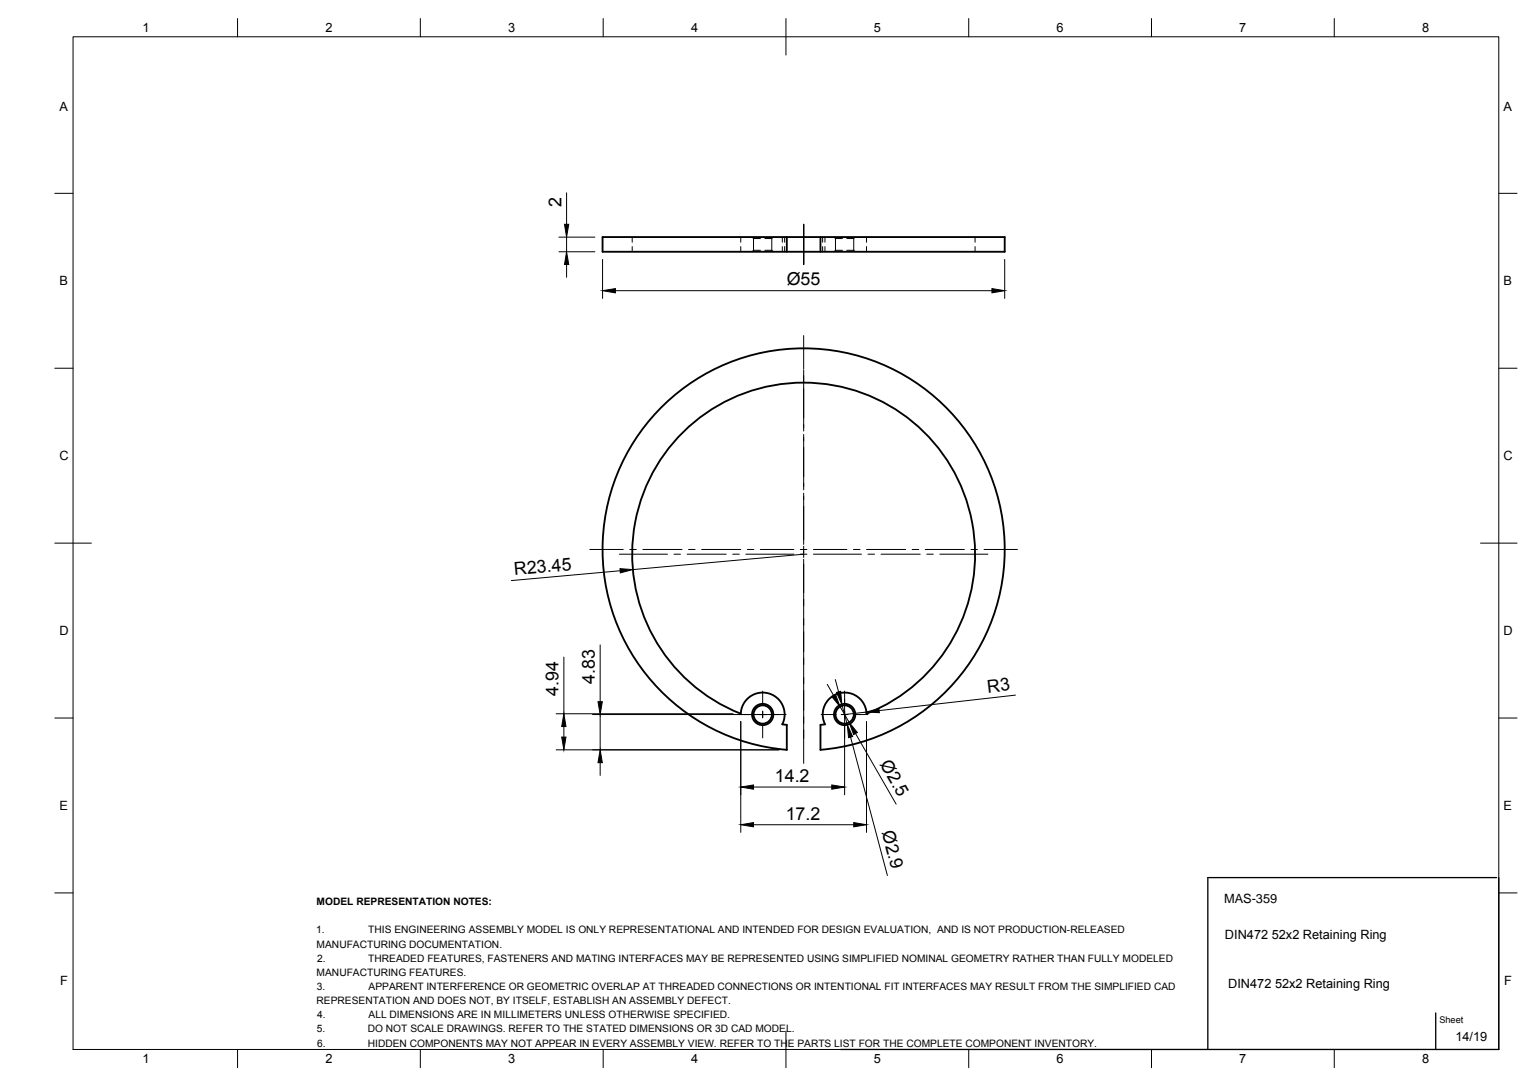
ISO-10303-21;
HEADER;
/* Generated by software containing ST-Developer
 * from STEP Tools, Inc. (www.steptools.com) 
 */

FILE_DESCRIPTION(
/* description */ (''),
/* implementation_level */ '2;1');

FILE_NAME(
/* name */ 'DIN472 52x2 Retaining Ring.step',
/* time_stamp */ '2026-10-15T14:25:16-07:00',
/* author */ (''),
/* organization */ (''),
/* preprocessor_version */ 'ST-DEVELOPER v20.2',
/* originating_system */ 'Autodesk Translation Framework v15.15.0.0',
/* authorisation */ '');

FILE_SCHEMA (('AUTOMOTIVE_DESIGN { 1 0 10303 214 3 1 1 }'));
ENDSEC;

DATA;
#10=MECHANICAL_DESIGN_GEOMETRIC_PRESENTATION_REPRESENTATION('',(#337),#86429);
#301=SHAPE_REPRESENTATION_RELATIONSHIP('SRR','None',#86516,#319);
#319=ADVANCED_BREP_SHAPE_REPRESENTATION('',(#355),#86425);
#337=STYLED_ITEM('',(#86615),#355);
#355=MANIFOLD_SOLID_BREP('Body1',#15627);
#1336=CONICAL_SURFACE('',#17085,0.135,0.785398163397449);
#1337=CONICAL_SURFACE('',#17098,0.135,0.785398163397448);
#1338=CONICAL_SURFACE('',#17108,0.135,0.785398163397449);
#1339=CONICAL_SURFACE('',#17112,0.135,0.785398163397448);
#1551=CYLINDRICAL_SURFACE('',#17088,0.125);
#1552=CYLINDRICAL_SURFACE('',#17110,0.125);
#1553=CYLINDRICAL_SURFACE('',#17115,2.345);
#1554=CYLINDRICAL_SURFACE('',#17116,0.3);
#1555=CYLINDRICAL_SURFACE('',#17117,2.345);
#1556=CYLINDRICAL_SURFACE('',#17118,0.3);
#1557=CYLINDRICAL_SURFACE('',#17119,2.345);
#1558=CYLINDRICAL_SURFACE('',#17120,2.75);
#1742=FACE_BOUND('',#4166,.T.);
#1743=FACE_BOUND('',#4167,.T.);
#1744=FACE_BOUND('',#4170,.T.);
#1745=FACE_BOUND('',#4171,.T.);
#2318=CIRCLE('',#17086,0.125);
#2319=CIRCLE('',#17087,0.145);
#2320=CIRCLE('',#17089,0.125);
#2321=CIRCLE('',#17091,2.75);
#2322=CIRCLE('',#17092,2.345);
#2323=CIRCLE('',#17093,0.3);
#2324=CIRCLE('',#17094,2.345);
#2325=CIRCLE('',#17095,0.3);
#2326=CIRCLE('',#17096,2.345);
#2327=CIRCLE('',#17097,0.145);
#2328=CIRCLE('',#17099,0.145);
#2329=CIRCLE('',#17101,2.345);
#2330=CIRCLE('',#17102,0.3);
#2331=CIRCLE('',#17103,2.345);
#2332=CIRCLE('',#17104,0.3);
#2333=CIRCLE('',#17105,2.345);
#2334=CIRCLE('',#17106,2.75);
#2335=CIRCLE('',#17107,0.145);
#2336=CIRCLE('',#17109,0.125);
#2337=CIRCLE('',#17111,0.125);
#3151=FACE_OUTER_BOUND('',#4163,.T.);
#3152=FACE_OUTER_BOUND('',#4164,.T.);
#3153=FACE_OUTER_BOUND('',#4165,.T.);
#3154=FACE_OUTER_BOUND('',#4168,.T.);
#3155=FACE_OUTER_BOUND('',#4169,.T.);
#3156=FACE_OUTER_BOUND('',#4172,.T.);
#3157=FACE_OUTER_BOUND('',#4173,.T.);
#3158=FACE_OUTER_BOUND('',#4174,.T.);
#3159=FACE_OUTER_BOUND('',#4175,.T.);
#3160=FACE_OUTER_BOUND('',#4176,.T.);
#3161=FACE_OUTER_BOUND('',#4177,.T.);
#3162=FACE_OUTER_BOUND('',#4178,.T.);
#3163=FACE_OUTER_BOUND('',#4179,.T.);
#3164=FACE_OUTER_BOUND('',#4180,.T.);
#3165=FACE_OUTER_BOUND('',#4181,.T.);
#3166=FACE_OUTER_BOUND('',#4182,.T.);
#4163=EDGE_LOOP('',(#13717,#13718,#13719,#13720));
#4164=EDGE_LOOP('',(#13721,#13722,#13723,#13724));
#4165=EDGE_LOOP('',(#13725,#13726,#13727,#13728,#13729,#13730,#13731,#13732));
#4166=EDGE_LOOP('',(#13733));
#4167=EDGE_LOOP('',(#13734));
#4168=EDGE_LOOP('',(#13735,#13736,#13737,#13738));
#4169=EDGE_LOOP('',(#13739,#13740,#13741,#13742,#13743,#13744,#13745,#13746));
#4170=EDGE_LOOP('',(#13747));
#4171=EDGE_LOOP('',(#13748));
#4172=EDGE_LOOP('',(#13749,#13750,#13751,#13752));
#4173=EDGE_LOOP('',(#13753,#13754,#13755,#13756));
#4174=EDGE_LOOP('',(#13757,#13758,#13759,#13760));
#4175=EDGE_LOOP('',(#13761,#13762,#13763,#13764));
#4176=EDGE_LOOP('',(#13765,#13766,#13767,#13768));
#4177=EDGE_LOOP('',(#13769,#13770,#13771,#13772));
#4178=EDGE_LOOP('',(#13773,#13774,#13775,#13776));
#4179=EDGE_LOOP('',(#13777,#13778,#13779,#13780));
#4180=EDGE_LOOP('',(#13781,#13782,#13783,#13784));
#4181=EDGE_LOOP('',(#13785,#13786,#13787,#13788));
#4182=EDGE_LOOP('',(#13789,#13790,#13791,#13792));
#5049=LINE('',#66556,#5909);
#5050=LINE('',#66560,#5910);
#5051=LINE('',#66565,#5911);
#5052=LINE('',#66569,#5912);
#5053=LINE('',#66583,#5913);
#5054=LINE('',#66588,#5914);
#5055=LINE('',#66600,#5915);
#5056=LINE('',#66607,#5916);
#5057=LINE('',#66610,#5917);
#5058=LINE('',#66613,#5918);
#5059=LINE('',#66615,#5919);
#5060=LINE('',#66616,#5920);
#5061=LINE('',#66618,#5921);
#5062=LINE('',#66619,#5922);
#5063=LINE('',#66621,#5923);
#5064=LINE('',#66623,#5924);
#5065=LINE('',#66625,#5925);
#5066=LINE('',#66627,#5926);
#5909=VECTOR('',#20568,0.135);
#5910=VECTOR('',#20573,0.125);
#5911=VECTOR('',#20578,1.);
#5912=VECTOR('',#20581,1.);
#5913=VECTOR('',#20596,0.135);
#5914=VECTOR('',#20601,1.);
#5915=VECTOR('',#20612,1.);
#5916=VECTOR('',#20621,0.135);
#5917=VECTOR('',#20624,0.125);
#5918=VECTOR('',#20629,0.135);
#5919=VECTOR('',#20632,1.);
#5920=VECTOR('',#20633,1.);
#5921=VECTOR('',#20636,1.);
#5922=VECTOR('',#20637,1.);
#5923=VECTOR('',#20640,1.);
#5924=VECTOR('',#20643,1.);
#5925=VECTOR('',#20646,1.);
#5926=VECTOR('',#20649,1.);
#7266=VERTEX_POINT('',#66553);
#7267=VERTEX_POINT('',#66555);
#7268=VERTEX_POINT('',#66559);
#7269=VERTEX_POINT('',#66563);
#7270=VERTEX_POINT('',#66564);
#7271=VERTEX_POINT('',#66566);
#7272=VERTEX_POINT('',#66568);
#7273=VERTEX_POINT('',#66570);
#7274=VERTEX_POINT('',#66572);
#7275=VERTEX_POINT('',#66574);
#7276=VERTEX_POINT('',#66576);
#7277=VERTEX_POINT('',#66579);
#7278=VERTEX_POINT('',#66582);
#7279=VERTEX_POINT('',#66586);
#7280=VERTEX_POINT('',#66587);
#7281=VERTEX_POINT('',#66589);
#7282=VERTEX_POINT('',#66591);
#7283=VERTEX_POINT('',#66593);
#7284=VERTEX_POINT('',#66595);
#7285=VERTEX_POINT('',#66597);
#7286=VERTEX_POINT('',#66599);
#7287=VERTEX_POINT('',#66602);
#7288=VERTEX_POINT('',#66605);
#7289=VERTEX_POINT('',#66609);
#9480=EDGE_CURVE('',#7266,#7266,#2318,.T.);
#9481=EDGE_CURVE('',#7266,#7267,#5049,.T.);
#9482=EDGE_CURVE('',#7267,#7267,#2319,.T.);
#9483=EDGE_CURVE('',#7266,#7268,#5050,.T.);
#9484=EDGE_CURVE('',#7268,#7268,#2320,.T.);
#9485=EDGE_CURVE('',#7269,#7270,#5051,.T.);
#9486=EDGE_CURVE('',#7271,#7270,#2321,.T.);
#9487=EDGE_CURVE('',#7271,#7272,#5052,.T.);
#9488=EDGE_CURVE('',#7273,#7272,#2322,.T.);
#9489=EDGE_CURVE('',#7274,#7273,#2323,.T.);
#9490=EDGE_CURVE('',#7275,#7274,#2324,.T.);
#9491=EDGE_CURVE('',#7276,#7275,#2325,.T.);
#9492=EDGE_CURVE('',#7269,#7276,#2326,.T.);
#9493=EDGE_CURVE('',#7277,#7277,#2327,.T.);
#9494=EDGE_CURVE('',#7268,#7278,#5053,.T.);
#9495=EDGE_CURVE('',#7278,#7278,#2328,.T.);
#9496=EDGE_CURVE('',#7279,#7280,#5054,.T.);
#9497=EDGE_CURVE('',#7280,#7281,#2329,.T.);
#9498=EDGE_CURVE('',#7281,#7282,#2330,.T.);
#9499=EDGE_CURVE('',#7282,#7283,#2331,.T.);
#9500=EDGE_CURVE('',#7283,#7284,#2332,.T.);
#9501=EDGE_CURVE('',#7284,#7285,#2333,.T.);
#9502=EDGE_CURVE('',#7285,#7286,#5055,.T.);
#9503=EDGE_CURVE('',#7286,#7279,#2334,.T.);
#9504=EDGE_CURVE('',#7287,#7287,#2335,.T.);
#9505=EDGE_CURVE('',#7288,#7288,#2336,.T.);
#9506=EDGE_CURVE('',#7288,#7277,#5056,.T.);
#9507=EDGE_CURVE('',#7288,#7289,#5057,.T.);
#9508=EDGE_CURVE('',#7289,#7289,#2337,.T.);
#9509=EDGE_CURVE('',#7289,#7287,#5058,.T.);
#9510=EDGE_CURVE('',#7272,#7285,#5059,.T.);
#9511=EDGE_CURVE('',#7286,#7271,#5060,.T.);
#9512=EDGE_CURVE('',#7280,#7269,#5061,.T.);
#9513=EDGE_CURVE('',#7270,#7279,#5062,.T.);
#9514=EDGE_CURVE('',#7273,#7284,#5063,.T.);
#9515=EDGE_CURVE('',#7274,#7283,#5064,.T.);
#9516=EDGE_CURVE('',#7275,#7282,#5065,.T.);
#9517=EDGE_CURVE('',#7276,#7281,#5066,.T.);
#13717=ORIENTED_EDGE('',*,*,#9480,.T.);
#13718=ORIENTED_EDGE('',*,*,#9481,.T.);
#13719=ORIENTED_EDGE('',*,*,#9482,.T.);
#13720=ORIENTED_EDGE('',*,*,#9481,.F.);
#13721=ORIENTED_EDGE('',*,*,#9480,.F.);
#13722=ORIENTED_EDGE('',*,*,#9483,.T.);
#13723=ORIENTED_EDGE('',*,*,#9484,.F.);
#13724=ORIENTED_EDGE('',*,*,#9483,.F.);
#13725=ORIENTED_EDGE('',*,*,#9485,.T.);
#13726=ORIENTED_EDGE('',*,*,#9486,.F.);
#13727=ORIENTED_EDGE('',*,*,#9487,.T.);
#13728=ORIENTED_EDGE('',*,*,#9488,.F.);
#13729=ORIENTED_EDGE('',*,*,#9489,.F.);
#13730=ORIENTED_EDGE('',*,*,#9490,.F.);
#13731=ORIENTED_EDGE('',*,*,#9491,.F.);
#13732=ORIENTED_EDGE('',*,*,#9492,.F.);
#13733=ORIENTED_EDGE('',*,*,#9493,.F.);
#13734=ORIENTED_EDGE('',*,*,#9482,.F.);
#13735=ORIENTED_EDGE('',*,*,#9484,.T.);
#13736=ORIENTED_EDGE('',*,*,#9494,.T.);
#13737=ORIENTED_EDGE('',*,*,#9495,.T.);
#13738=ORIENTED_EDGE('',*,*,#9494,.F.);
#13739=ORIENTED_EDGE('',*,*,#9496,.T.);
#13740=ORIENTED_EDGE('',*,*,#9497,.T.);
#13741=ORIENTED_EDGE('',*,*,#9498,.T.);
#13742=ORIENTED_EDGE('',*,*,#9499,.T.);
#13743=ORIENTED_EDGE('',*,*,#9500,.T.);
#13744=ORIENTED_EDGE('',*,*,#9501,.T.);
#13745=ORIENTED_EDGE('',*,*,#9502,.T.);
#13746=ORIENTED_EDGE('',*,*,#9503,.T.);
#13747=ORIENTED_EDGE('',*,*,#9504,.F.);
#13748=ORIENTED_EDGE('',*,*,#9495,.F.);
#13749=ORIENTED_EDGE('',*,*,#9505,.T.);
#13750=ORIENTED_EDGE('',*,*,#9506,.T.);
#13751=ORIENTED_EDGE('',*,*,#9493,.T.);
#13752=ORIENTED_EDGE('',*,*,#9506,.F.);
#13753=ORIENTED_EDGE('',*,*,#9505,.F.);
#13754=ORIENTED_EDGE('',*,*,#9507,.T.);
#13755=ORIENTED_EDGE('',*,*,#9508,.F.);
#13756=ORIENTED_EDGE('',*,*,#9507,.F.);
#13757=ORIENTED_EDGE('',*,*,#9508,.T.);
#13758=ORIENTED_EDGE('',*,*,#9509,.T.);
#13759=ORIENTED_EDGE('',*,*,#9504,.T.);
#13760=ORIENTED_EDGE('',*,*,#9509,.F.);
#13761=ORIENTED_EDGE('',*,*,#9510,.F.);
#13762=ORIENTED_EDGE('',*,*,#9487,.F.);
#13763=ORIENTED_EDGE('',*,*,#9511,.F.);
#13764=ORIENTED_EDGE('',*,*,#9502,.F.);
#13765=ORIENTED_EDGE('',*,*,#9512,.F.);
#13766=ORIENTED_EDGE('',*,*,#9496,.F.);
#13767=ORIENTED_EDGE('',*,*,#9513,.F.);
#13768=ORIENTED_EDGE('',*,*,#9485,.F.);
#13769=ORIENTED_EDGE('',*,*,#9510,.T.);
#13770=ORIENTED_EDGE('',*,*,#9501,.F.);
#13771=ORIENTED_EDGE('',*,*,#9514,.F.);
#13772=ORIENTED_EDGE('',*,*,#9488,.T.);
#13773=ORIENTED_EDGE('',*,*,#9489,.T.);
#13774=ORIENTED_EDGE('',*,*,#9514,.T.);
#13775=ORIENTED_EDGE('',*,*,#9500,.F.);
#13776=ORIENTED_EDGE('',*,*,#9515,.F.);
#13777=ORIENTED_EDGE('',*,*,#9490,.T.);
#13778=ORIENTED_EDGE('',*,*,#9515,.T.);
#13779=ORIENTED_EDGE('',*,*,#9499,.F.);
#13780=ORIENTED_EDGE('',*,*,#9516,.F.);
#13781=ORIENTED_EDGE('',*,*,#9491,.T.);
#13782=ORIENTED_EDGE('',*,*,#9516,.T.);
#13783=ORIENTED_EDGE('',*,*,#9498,.F.);
#13784=ORIENTED_EDGE('',*,*,#9517,.F.);
#13785=ORIENTED_EDGE('',*,*,#9512,.T.);
#13786=ORIENTED_EDGE('',*,*,#9492,.T.);
#13787=ORIENTED_EDGE('',*,*,#9517,.T.);
#13788=ORIENTED_EDGE('',*,*,#9497,.F.);
#13789=ORIENTED_EDGE('',*,*,#9513,.T.);
#13790=ORIENTED_EDGE('',*,*,#9503,.F.);
#13791=ORIENTED_EDGE('',*,*,#9511,.T.);
#13792=ORIENTED_EDGE('',*,*,#9486,.T.);
#14709=PLANE('',#17090);
#14710=PLANE('',#17100);
#14711=PLANE('',#17113);
#14712=PLANE('',#17114);
#15507=ADVANCED_FACE('',(#3151),#1336,.F.);
#15508=ADVANCED_FACE('',(#3152),#1551,.F.);
#15509=ADVANCED_FACE('',(#3153,#1742,#1743),#14709,.F.);
#15510=ADVANCED_FACE('',(#3154),#1337,.F.);
#15511=ADVANCED_FACE('',(#3155,#1744,#1745),#14710,.T.);
#15512=ADVANCED_FACE('',(#3156),#1338,.F.);
#15513=ADVANCED_FACE('',(#3157),#1552,.F.);
#15514=ADVANCED_FACE('',(#3158),#1339,.F.);
#15515=ADVANCED_FACE('',(#3159),#14711,.F.);
#15516=ADVANCED_FACE('',(#3160),#14712,.F.);
#15517=ADVANCED_FACE('',(#3161),#1553,.F.);
#15518=ADVANCED_FACE('',(#3162),#1554,.T.);
#15519=ADVANCED_FACE('',(#3163),#1555,.F.);
#15520=ADVANCED_FACE('',(#3164),#1556,.T.);
#15521=ADVANCED_FACE('',(#3165),#1557,.F.);
#15522=ADVANCED_FACE('',(#3166),#1558,.T.);
#15627=CLOSED_SHELL('',(#15507,#15508,#15509,#15510,#15511,#15512,#15513,
#15514,#15515,#15516,#15517,#15518,#15519,#15520,#15521,#15522));
#17084=AXIS2_PLACEMENT_3D('',#66551,#20562,#20563);
#17085=AXIS2_PLACEMENT_3D('',#66552,#20564,#20565);
#17086=AXIS2_PLACEMENT_3D('',#66554,#20566,#20567);
#17087=AXIS2_PLACEMENT_3D('',#66557,#20569,#20570);
#17088=AXIS2_PLACEMENT_3D('',#66558,#20571,#20572);
#17089=AXIS2_PLACEMENT_3D('',#66561,#20574,#20575);
#17090=AXIS2_PLACEMENT_3D('',#66562,#20576,#20577);
#17091=AXIS2_PLACEMENT_3D('',#66567,#20579,#20580);
#17092=AXIS2_PLACEMENT_3D('',#66571,#20582,#20583);
#17093=AXIS2_PLACEMENT_3D('',#66573,#20584,#20585);
#17094=AXIS2_PLACEMENT_3D('',#66575,#20586,#20587);
#17095=AXIS2_PLACEMENT_3D('',#66577,#20588,#20589);
#17096=AXIS2_PLACEMENT_3D('',#66578,#20590,#20591);
#17097=AXIS2_PLACEMENT_3D('',#66580,#20592,#20593);
#17098=AXIS2_PLACEMENT_3D('',#66581,#20594,#20595);
#17099=AXIS2_PLACEMENT_3D('',#66584,#20597,#20598);
#17100=AXIS2_PLACEMENT_3D('',#66585,#20599,#20600);
#17101=AXIS2_PLACEMENT_3D('',#66590,#20602,#20603);
#17102=AXIS2_PLACEMENT_3D('',#66592,#20604,#20605);
#17103=AXIS2_PLACEMENT_3D('',#66594,#20606,#20607);
#17104=AXIS2_PLACEMENT_3D('',#66596,#20608,#20609);
#17105=AXIS2_PLACEMENT_3D('',#66598,#20610,#20611);
#17106=AXIS2_PLACEMENT_3D('',#66601,#20613,#20614);
#17107=AXIS2_PLACEMENT_3D('',#66603,#20615,#20616);
#17108=AXIS2_PLACEMENT_3D('',#66604,#20617,#20618);
#17109=AXIS2_PLACEMENT_3D('',#66606,#20619,#20620);
#17110=AXIS2_PLACEMENT_3D('',#66608,#20622,#20623);
#17111=AXIS2_PLACEMENT_3D('',#66611,#20625,#20626);
#17112=AXIS2_PLACEMENT_3D('',#66612,#20627,#20628);
#17113=AXIS2_PLACEMENT_3D('',#66614,#20630,#20631);
#17114=AXIS2_PLACEMENT_3D('',#66617,#20634,#20635);
#17115=AXIS2_PLACEMENT_3D('',#66620,#20638,#20639);
#17116=AXIS2_PLACEMENT_3D('',#66622,#20641,#20642);
#17117=AXIS2_PLACEMENT_3D('',#66624,#20644,#20645);
#17118=AXIS2_PLACEMENT_3D('',#66626,#20647,#20648);
#17119=AXIS2_PLACEMENT_3D('',#66628,#20650,#20651);
#17120=AXIS2_PLACEMENT_3D('',#66629,#20652,#20653);
#20562=DIRECTION('axis',(0.,0.,1.));
#20563=DIRECTION('refdir',(1.,0.,0.));
#20564=DIRECTION('center_axis',(0.,0.,-1.));
#20565=DIRECTION('ref_axis',(1.,0.,0.));
#20566=DIRECTION('center_axis',(0.,0.,1.));
#20567=DIRECTION('ref_axis',(1.,0.,0.));
#20568=DIRECTION('',(-0.707106781186548,8.65956056235494E-17,-0.707106781186547));
#20569=DIRECTION('center_axis',(0.,0.,-1.));
#20570=DIRECTION('ref_axis',(1.,0.,0.));
#20571=DIRECTION('center_axis',(0.,0.,1.));
#20572=DIRECTION('ref_axis',(1.,0.,0.));
#20573=DIRECTION('',(0.,0.,1.));
#20574=DIRECTION('center_axis',(0.,0.,-1.));
#20575=DIRECTION('ref_axis',(1.,0.,0.));
#20576=DIRECTION('center_axis',(0.,0.,1.));
#20577=DIRECTION('ref_axis',(1.,0.,0.));
#20578=DIRECTION('',(0.,1.,0.));
#20579=DIRECTION('center_axis',(0.,0.,1.));
#20580=DIRECTION('ref_axis',(1.,0.,0.));
#20581=DIRECTION('',(0.,-1.,0.));
#20582=DIRECTION('center_axis',(0.,0.,-1.));
#20583=DIRECTION('ref_axis',(1.,0.,0.));
#20584=DIRECTION('center_axis',(0.,0.,1.));
#20585=DIRECTION('ref_axis',(1.,0.,0.));
#20586=DIRECTION('center_axis',(0.,0.,-1.));
#20587=DIRECTION('ref_axis',(1.,0.,0.));
#20588=DIRECTION('center_axis',(0.,0.,1.));
#20589=DIRECTION('ref_axis',(1.,0.,0.));
#20590=DIRECTION('center_axis',(0.,0.,-1.));
#20591=DIRECTION('ref_axis',(1.,0.,0.));
#20592=DIRECTION('center_axis',(0.,0.,-1.));
#20593=DIRECTION('ref_axis',(1.,0.,0.));
#20594=DIRECTION('center_axis',(0.,0.,1.));
#20595=DIRECTION('ref_axis',(1.,0.,0.));
#20596=DIRECTION('',(-0.707106781186547,-8.65956056235493E-17,0.707106781186548));
#20597=DIRECTION('center_axis',(0.,0.,1.));
#20598=DIRECTION('ref_axis',(1.,0.,0.));
#20599=DIRECTION('center_axis',(0.,0.,1.));
#20600=DIRECTION('ref_axis',(1.,0.,0.));
#20601=DIRECTION('',(0.,-1.,0.));
#20602=DIRECTION('center_axis',(0.,0.,-1.));
#20603=DIRECTION('ref_axis',(1.,0.,0.));
#20604=DIRECTION('center_axis',(0.,0.,1.));
#20605=DIRECTION('ref_axis',(1.,0.,0.));
#20606=DIRECTION('center_axis',(0.,0.,-1.));
#20607=DIRECTION('ref_axis',(1.,0.,0.));
#20608=DIRECTION('center_axis',(0.,0.,1.));
#20609=DIRECTION('ref_axis',(1.,0.,0.));
#20610=DIRECTION('center_axis',(0.,0.,-1.));
#20611=DIRECTION('ref_axis',(1.,0.,0.));
#20612=DIRECTION('',(0.,1.,0.));
#20613=DIRECTION('center_axis',(0.,0.,1.));
#20614=DIRECTION('ref_axis',(1.,0.,0.));
#20615=DIRECTION('center_axis',(0.,0.,1.));
#20616=DIRECTION('ref_axis',(1.,0.,0.));
#20617=DIRECTION('center_axis',(0.,0.,-1.));
#20618=DIRECTION('ref_axis',(1.,0.,0.));
#20619=DIRECTION('center_axis',(0.,0.,1.));
#20620=DIRECTION('ref_axis',(1.,0.,0.));
#20621=DIRECTION('',(-0.707106781186548,8.65956056235494E-17,-0.707106781186547));
#20622=DIRECTION('center_axis',(0.,0.,1.));
#20623=DIRECTION('ref_axis',(1.,0.,0.));
#20624=DIRECTION('',(0.,0.,1.));
#20625=DIRECTION('center_axis',(0.,0.,-1.));
#20626=DIRECTION('ref_axis',(1.,0.,0.));
#20627=DIRECTION('center_axis',(0.,0.,1.));
#20628=DIRECTION('ref_axis',(1.,0.,0.));
#20629=DIRECTION('',(-0.707106781186547,-8.65956056235493E-17,0.707106781186548));
#20630=DIRECTION('center_axis',(-1.,0.,0.));
#20631=DIRECTION('ref_axis',(0.,-1.,0.));
#20632=DIRECTION('',(0.,0.,1.));
#20633=DIRECTION('',(0.,0.,-1.));
#20634=DIRECTION('center_axis',(1.,0.,0.));
#20635=DIRECTION('ref_axis',(0.,1.,0.));
#20636=DIRECTION('',(0.,0.,-1.));
#20637=DIRECTION('',(0.,0.,1.));
#20638=DIRECTION('center_axis',(0.,0.,1.));
#20639=DIRECTION('ref_axis',(1.,0.,0.));
#20640=DIRECTION('',(0.,0.,1.));
#20641=DIRECTION('center_axis',(0.,0.,1.));
#20642=DIRECTION('ref_axis',(1.,0.,0.));
#20643=DIRECTION('',(0.,0.,1.));
#20644=DIRECTION('center_axis',(0.,0.,1.));
#20645=DIRECTION('ref_axis',(-1.83697019872103E-16,-1.,0.));
#20646=DIRECTION('',(0.,0.,1.));
#20647=DIRECTION('center_axis',(0.,0.,1.));
#20648=DIRECTION('ref_axis',(-0.247524504876091,-0.96888163337213,0.));
#20649=DIRECTION('',(0.,0.,1.));
#20650=DIRECTION('center_axis',(0.,0.,1.));
#20651=DIRECTION('ref_axis',(1.,0.,0.));
#20652=DIRECTION('center_axis',(0.,0.,1.));
#20653=DIRECTION('ref_axis',(6.12323399573677E-17,-1.,0.));
#66551=CARTESIAN_POINT('',(0.,0.,0.));
#66552=CARTESIAN_POINT('Origin',(-0.56,2.257,0.01));
#66553=CARTESIAN_POINT('',(-0.685,2.257,0.02));
#66554=CARTESIAN_POINT('Origin',(-0.56,2.257,0.02));
#66555=CARTESIAN_POINT('',(-0.705,2.257,0.));
#66556=CARTESIAN_POINT('',(-0.695,2.257,0.01));
#66557=CARTESIAN_POINT('Origin',(-0.56,2.257,0.));
#66558=CARTESIAN_POINT('Origin',(-0.56,2.257,0.));
#66559=CARTESIAN_POINT('',(-0.685,2.257,0.18));
#66560=CARTESIAN_POINT('',(-0.685,2.257,0.));
#66561=CARTESIAN_POINT('Origin',(-0.56,2.257,0.18));
#66562=CARTESIAN_POINT('Origin',(0.,0.,0.));
#66563=CARTESIAN_POINT('',(0.23,2.39869342459544,0.));
#66564=CARTESIAN_POINT('',(0.23,2.74036493920062,0.));
#66565=CARTESIAN_POINT('',(0.23,0.9,0.));
#66566=CARTESIAN_POINT('',(-0.23,2.74036493920062,0.));
#66567=CARTESIAN_POINT('Origin',(0.,0.,0.));
#66568=CARTESIAN_POINT('',(-0.23,2.39869342459544,0.));
#66569=CARTESIAN_POINT('',(-0.23,1.45,0.));
#66570=CARTESIAN_POINT('',(-0.291967181462275,2.39175313794759,0.));
#66571=CARTESIAN_POINT('Origin',(0.,0.065,0.));
#66572=CARTESIAN_POINT('',(-0.859822464806605,2.24668062030488,0.));
#66573=CARTESIAN_POINT('Origin',(-0.56,2.257,0.));
#66574=CARTESIAN_POINT('',(0.859822464806605,2.24668062030488,0.));
#66575=CARTESIAN_POINT('Origin',(0.,0.065,0.));
#66576=CARTESIAN_POINT('',(0.291967181462275,2.39175313794759,0.));
#66577=CARTESIAN_POINT('Origin',(0.56,2.257,0.));
#66578=CARTESIAN_POINT('Origin',(0.,0.065,0.));
#66579=CARTESIAN_POINT('',(0.415,2.257,0.));
#66580=CARTESIAN_POINT('Origin',(0.56,2.257,0.));
#66581=CARTESIAN_POINT('Origin',(-0.56,2.257,0.19));
#66582=CARTESIAN_POINT('',(-0.705,2.257,0.2));
#66583=CARTESIAN_POINT('',(-0.695,2.257,0.19));
#66584=CARTESIAN_POINT('Origin',(-0.56,2.257,0.2));
#66585=CARTESIAN_POINT('Origin',(0.,0.,0.2));
#66586=CARTESIAN_POINT('',(0.23,2.74036493920062,0.2));
#66587=CARTESIAN_POINT('',(0.23,2.39869342459544,0.2));
#66588=CARTESIAN_POINT('',(0.23,0.9,0.2));
#66589=CARTESIAN_POINT('',(0.291967181462275,2.39175313794759,0.2));
#66590=CARTESIAN_POINT('Origin',(0.,0.065,0.2));
#66591=CARTESIAN_POINT('',(0.859822464806605,2.24668062030488,0.2));
#66592=CARTESIAN_POINT('Origin',(0.56,2.257,0.2));
#66593=CARTESIAN_POINT('',(-0.859822464806605,2.24668062030488,0.2));
#66594=CARTESIAN_POINT('Origin',(0.,0.065,0.2));
#66595=CARTESIAN_POINT('',(-0.291967181462275,2.39175313794759,0.2));
#66596=CARTESIAN_POINT('Origin',(-0.56,2.257,0.2));
#66597=CARTESIAN_POINT('',(-0.23,2.39869342459544,0.2));
#66598=CARTESIAN_POINT('Origin',(0.,0.065,0.2));
#66599=CARTESIAN_POINT('',(-0.23,2.74036493920062,0.2));
#66600=CARTESIAN_POINT('',(-0.23,1.45,0.2));
#66601=CARTESIAN_POINT('Origin',(0.,0.,0.2));
#66602=CARTESIAN_POINT('',(0.415,2.257,0.2));
#66603=CARTESIAN_POINT('Origin',(0.56,2.257,0.2));
#66604=CARTESIAN_POINT('Origin',(0.56,2.257,0.01));
#66605=CARTESIAN_POINT('',(0.435,2.257,0.02));
#66606=CARTESIAN_POINT('Origin',(0.56,2.257,0.02));
#66607=CARTESIAN_POINT('',(0.425,2.257,0.01));
#66608=CARTESIAN_POINT('Origin',(0.56,2.257,0.));
#66609=CARTESIAN_POINT('',(0.435,2.257,0.18));
#66610=CARTESIAN_POINT('',(0.435,2.257,0.));
#66611=CARTESIAN_POINT('Origin',(0.56,2.257,0.18));
#66612=CARTESIAN_POINT('Origin',(0.56,2.257,0.19));
#66613=CARTESIAN_POINT('',(0.425,2.257,0.19));
#66614=CARTESIAN_POINT('Origin',(-0.23,2.9,0.));
#66615=CARTESIAN_POINT('',(-0.23,2.39869342459544,0.));
#66616=CARTESIAN_POINT('',(-0.23,2.74036493920062,0.));
#66617=CARTESIAN_POINT('Origin',(0.23,1.8,0.));
#66618=CARTESIAN_POINT('',(0.23,2.39869342459544,0.));
#66619=CARTESIAN_POINT('',(0.23,2.74036493920062,0.));
#66620=CARTESIAN_POINT('Origin',(0.,0.065,0.));
#66621=CARTESIAN_POINT('',(-0.291967181462275,2.39175313794759,0.));
#66622=CARTESIAN_POINT('Origin',(-0.56,2.257,0.));
#66623=CARTESIAN_POINT('',(-0.859822464806605,2.24668062030488,0.));
#66624=CARTESIAN_POINT('Origin',(0.,0.065,0.));
#66625=CARTESIAN_POINT('',(0.859822464806605,2.24668062030488,0.));
#66626=CARTESIAN_POINT('Origin',(0.56,2.257,0.));
#66627=CARTESIAN_POINT('',(0.291967181462275,2.39175313794759,0.));
#66628=CARTESIAN_POINT('Origin',(0.,0.065,0.));
#66629=CARTESIAN_POINT('Origin',(0.,0.,0.));
#86405=UNCERTAINTY_MEASURE_WITH_UNIT(LENGTH_MEASURE(0.001),#86430,
'DISTANCE_ACCURACY_VALUE',
'Maximum model space distance between geometric entities at asserted c
onnectivities');
#86409=UNCERTAINTY_MEASURE_WITH_UNIT(LENGTH_MEASURE(0.001),#86430,
'DISTANCE_ACCURACY_VALUE',
'Maximum model space distance between geometric entities at asserted c
onnectivities');
#86425=(
GEOMETRIC_REPRESENTATION_CONTEXT(3)
GLOBAL_UNCERTAINTY_ASSIGNED_CONTEXT((#86405))
GLOBAL_UNIT_ASSIGNED_CONTEXT((#86430,#86432,#86433))
REPRESENTATION_CONTEXT('','3D')
);
#86429=(
GEOMETRIC_REPRESENTATION_CONTEXT(3)
GLOBAL_UNCERTAINTY_ASSIGNED_CONTEXT((#86409))
GLOBAL_UNIT_ASSIGNED_CONTEXT((#86430,#86432,#86433))
REPRESENTATION_CONTEXT('','3D')
);
#86430=(
LENGTH_UNIT()
NAMED_UNIT(*)
SI_UNIT(.CENTI.,.METRE.)
);
#86432=(
NAMED_UNIT(*)
PLANE_ANGLE_UNIT()
SI_UNIT($,.RADIAN.)
);
#86433=(
NAMED_UNIT(*)
SI_UNIT($,.STERADIAN.)
SOLID_ANGLE_UNIT()
);
#86449=SHAPE_DEFINITION_REPRESENTATION(#86468,#86516);
#86468=PRODUCT_DEFINITION_SHAPE('',$,#86536);
#86516=SHAPE_REPRESENTATION('',(#17084),#86425);
#86520=PRODUCT_DEFINITION_CONTEXT('part definition',#86579,'design');
#86536=PRODUCT_DEFINITION('DIN472 52x2 Retaining Ring',
'DIN472 52x2 Retaining Ring',#86555,#86520);
#86555=PRODUCT_DEFINITION_FORMATION('',$,#86596);
#86579=APPLICATION_CONTEXT(
'Core Data for Automotive Mechanical Design Process');
#86580=PRODUCT_CONTEXT('part definition',#86579,'mechanical');
#86596=PRODUCT('DIN472 52x2 Retaining Ring',
'DIN472 52x2 Retaining Ring',$,(#86580));
#86615=PRESENTATION_STYLE_ASSIGNMENT((#86633));
#86633=SURFACE_STYLE_USAGE(.BOTH.,#86651);
#86651=SURFACE_SIDE_STYLE('',(#86669));
#86669=SURFACE_STYLE_FILL_AREA(#86687);
#86687=FILL_AREA_STYLE('Opaque(200,204,208)',(#86705));
#86705=FILL_AREA_STYLE_COLOUR('Opaque(200,204,208)',#86723);
#86723=COLOUR_RGB('Opaque(200,204,208)', 0.31764706, 0.68627451, 0.89019608);
ENDSEC;
END-ISO-10303-21;
